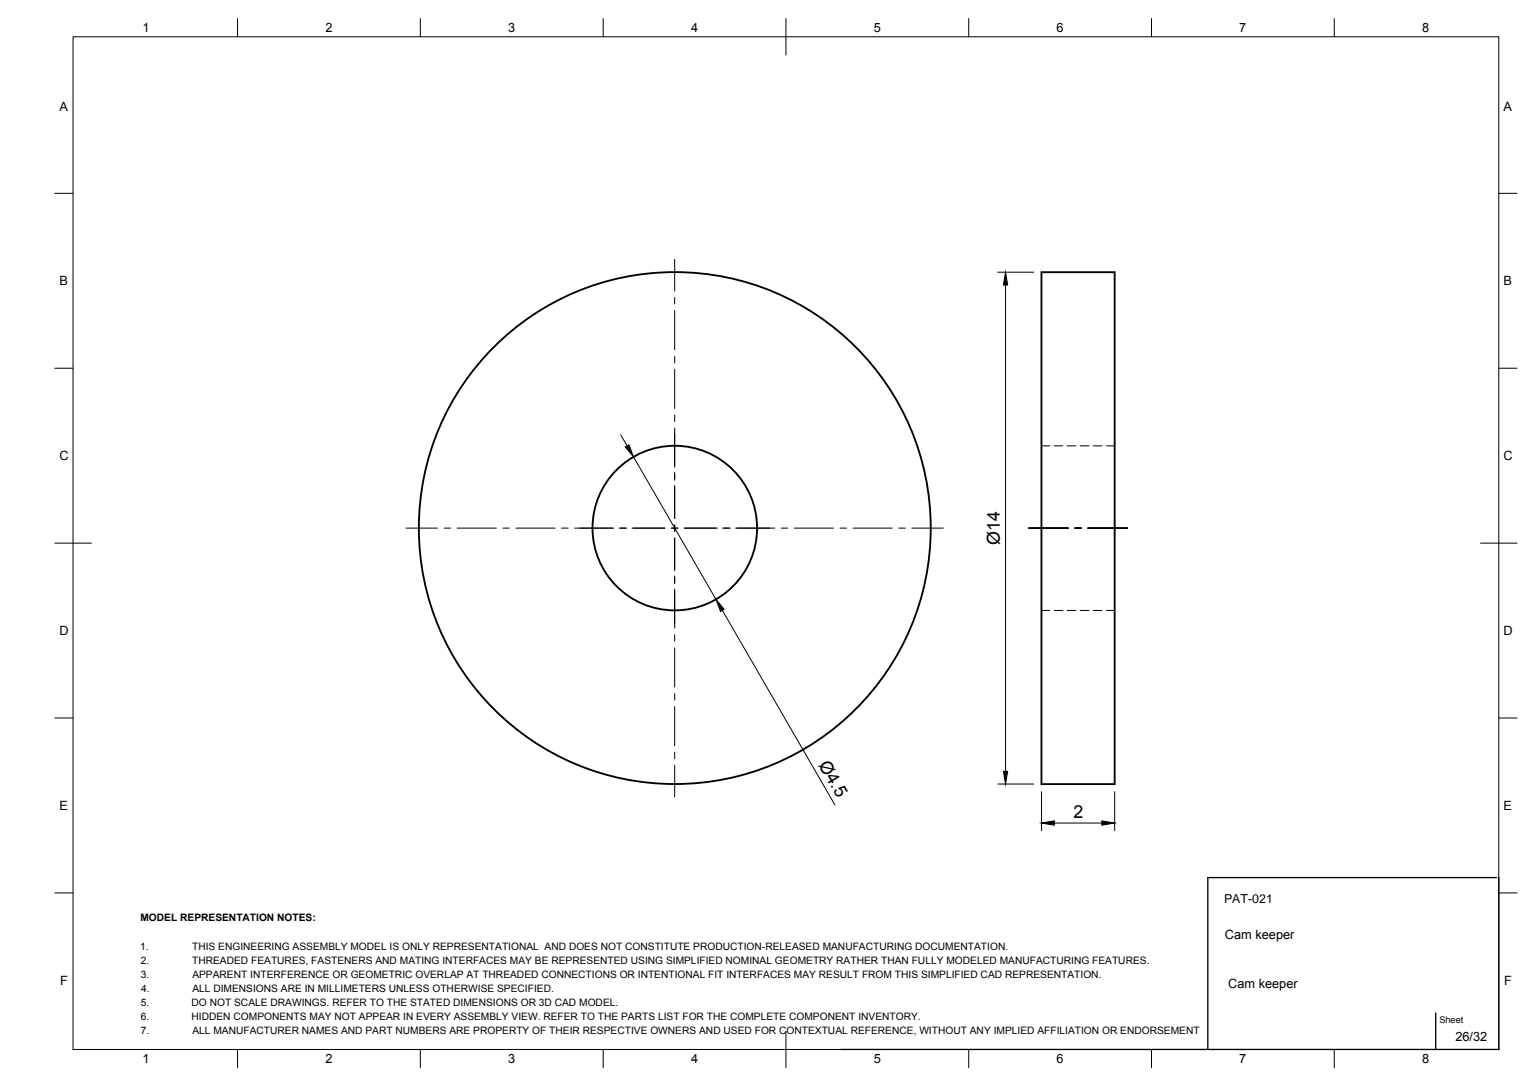
ISO-10303-21;
HEADER;
/* Generated by software containing ST-Developer
 * from STEP Tools, Inc. (www.steptools.com) 
 */

FILE_DESCRIPTION(
/* description */ ('Chain-less indexing wheel (Geneva) drive'),
/* implementation_level */ '2;1');

FILE_NAME(
/* name */ 'Cam keeper.step',
/* time_stamp */ '2026-10-28T03:25:22-07:00',
/* author */ (''),
/* organization */ (''),
/* preprocessor_version */ 'ST-DEVELOPER v20.2',
/* originating_system */ 'Autodesk Translation Framework v15.17.0.0',
/* authorisation */ '');

FILE_SCHEMA (('AUTOMOTIVE_DESIGN { 1 0 10303 214 3 1 1 }'));
ENDSEC;

DATA;
#10=MECHANICAL_DESIGN_GEOMETRIC_PRESENTATION_REPRESENTATION('',(#329),#10957);
#271=SHAPE_REPRESENTATION_RELATIONSHIP('SRR','None',#11086,#296);
#296=ADVANCED_BREP_SHAPE_REPRESENTATION('',(#361),#10949);
#329=STYLED_ITEM('',(#11273),#361);
#361=MANIFOLD_SOLID_BREP('Body1',#5726);
#451=FACE_BOUND('',#1299,.T.);
#452=FACE_BOUND('',#1301,.T.);
#585=PLANE('',#6514);
#586=PLANE('',#6515);
#879=FACE_OUTER_BOUND('',#1296,.T.);
#880=FACE_OUTER_BOUND('',#1297,.T.);
#881=FACE_OUTER_BOUND('',#1298,.T.);
#882=FACE_OUTER_BOUND('',#1300,.T.);
#1296=EDGE_LOOP('',(#4719,#4720,#4721,#4722));
#1297=EDGE_LOOP('',(#4723,#4724,#4725,#4726));
#1298=EDGE_LOOP('',(#4727));
#1299=EDGE_LOOP('',(#4728));
#1300=EDGE_LOOP('',(#4729));
#1301=EDGE_LOOP('',(#4730));
#1636=LINE('',#10193,#2010);
#1637=LINE('',#10199,#2011);
#2010=VECTOR('',#7962,0.225);
#2011=VECTOR('',#7969,0.7);
#2414=CIRCLE('',#6509,0.225);
#2415=CIRCLE('',#6510,0.225);
#2416=CIRCLE('',#6512,0.7);
#2417=CIRCLE('',#6513,0.7);
#2826=VERTEX_POINT('',#10190);
#2827=VERTEX_POINT('',#10192);
#2828=VERTEX_POINT('',#10196);
#2829=VERTEX_POINT('',#10198);
#3485=EDGE_CURVE('',#2826,#2826,#2414,.T.);
#3486=EDGE_CURVE('',#2826,#2827,#1636,.T.);
#3487=EDGE_CURVE('',#2827,#2827,#2415,.T.);
#3488=EDGE_CURVE('',#2828,#2828,#2416,.T.);
#3489=EDGE_CURVE('',#2828,#2829,#1637,.T.);
#3490=EDGE_CURVE('',#2829,#2829,#2417,.T.);
#4719=ORIENTED_EDGE('',*,*,#3485,.F.);
#4720=ORIENTED_EDGE('',*,*,#3486,.T.);
#4721=ORIENTED_EDGE('',*,*,#3487,.T.);
#4722=ORIENTED_EDGE('',*,*,#3486,.F.);
#4723=ORIENTED_EDGE('',*,*,#3488,.F.);
#4724=ORIENTED_EDGE('',*,*,#3489,.T.);
#4725=ORIENTED_EDGE('',*,*,#3490,.T.);
#4726=ORIENTED_EDGE('',*,*,#3489,.F.);
#4727=ORIENTED_EDGE('',*,*,#3488,.T.);
#4728=ORIENTED_EDGE('',*,*,#3485,.T.);
#4729=ORIENTED_EDGE('',*,*,#3490,.F.);
#4730=ORIENTED_EDGE('',*,*,#3487,.F.);
#5331=CYLINDRICAL_SURFACE('',#6508,0.225);
#5332=CYLINDRICAL_SURFACE('',#6511,0.7);
#5593=ADVANCED_FACE('',(#879),#5331,.F.);
#5594=ADVANCED_FACE('',(#880),#5332,.T.);
#5595=ADVANCED_FACE('',(#881,#451),#585,.T.);
#5596=ADVANCED_FACE('',(#882,#452),#586,.F.);
#5726=CLOSED_SHELL('',(#5593,#5594,#5595,#5596));
#6507=AXIS2_PLACEMENT_3D('',#10188,#7956,#7957);
#6508=AXIS2_PLACEMENT_3D('',#10189,#7958,#7959);
#6509=AXIS2_PLACEMENT_3D('',#10191,#7960,#7961);
#6510=AXIS2_PLACEMENT_3D('',#10194,#7963,#7964);
#6511=AXIS2_PLACEMENT_3D('',#10195,#7965,#7966);
#6512=AXIS2_PLACEMENT_3D('',#10197,#7967,#7968);
#6513=AXIS2_PLACEMENT_3D('',#10200,#7970,#7971);
#6514=AXIS2_PLACEMENT_3D('',#10201,#7972,#7973);
#6515=AXIS2_PLACEMENT_3D('',#10202,#7974,#7975);
#7956=DIRECTION('axis',(0.,0.,1.));
#7957=DIRECTION('refdir',(1.,0.,0.));
#7958=DIRECTION('center_axis',(0.,0.,1.));
#7959=DIRECTION('ref_axis',(1.,0.,0.));
#7960=DIRECTION('center_axis',(0.,0.,-1.));
#7961=DIRECTION('ref_axis',(1.,0.,0.));
#7962=DIRECTION('',(0.,0.,-1.));
#7963=DIRECTION('center_axis',(0.,0.,-1.));
#7964=DIRECTION('ref_axis',(1.,0.,0.));
#7965=DIRECTION('center_axis',(0.,0.,1.));
#7966=DIRECTION('ref_axis',(1.,0.,0.));
#7967=DIRECTION('center_axis',(0.,0.,1.));
#7968=DIRECTION('ref_axis',(1.,0.,0.));
#7969=DIRECTION('',(0.,0.,-1.));
#7970=DIRECTION('center_axis',(0.,0.,1.));
#7971=DIRECTION('ref_axis',(1.,0.,0.));
#7972=DIRECTION('center_axis',(0.,0.,1.));
#7973=DIRECTION('ref_axis',(1.,0.,0.));
#7974=DIRECTION('center_axis',(0.,0.,1.));
#7975=DIRECTION('ref_axis',(1.,0.,0.));
#10188=CARTESIAN_POINT('',(0.,0.,0.));
#10189=CARTESIAN_POINT('Origin',(0.,0.,6.8));
#10190=CARTESIAN_POINT('',(-0.225,-2.75545529808154E-17,7.));
#10191=CARTESIAN_POINT('Origin',(0.,0.,7.));
#10192=CARTESIAN_POINT('',(-0.225,-2.75545529808154E-17,6.8));
#10193=CARTESIAN_POINT('',(-0.225,-2.75545529808154E-17,6.8));
#10194=CARTESIAN_POINT('Origin',(0.,0.,6.8));
#10195=CARTESIAN_POINT('Origin',(0.,0.,6.8));
#10196=CARTESIAN_POINT('',(-0.7,-8.57252759403147E-17,7.));
#10197=CARTESIAN_POINT('Origin',(0.,0.,7.));
#10198=CARTESIAN_POINT('',(-0.7,-8.57252759403147E-17,6.8));
#10199=CARTESIAN_POINT('',(-0.7,-8.57252759403147E-17,6.8));
#10200=CARTESIAN_POINT('Origin',(0.,0.,6.8));
#10201=CARTESIAN_POINT('Origin',(0.,0.,7.));
#10202=CARTESIAN_POINT('Origin',(0.,0.,6.8));
#10918=UNCERTAINTY_MEASURE_WITH_UNIT(LENGTH_MEASURE(0.001),#10958,
'DISTANCE_ACCURACY_VALUE',
'Maximum model space distance between geometric entities at asserted c
onnectivities');
#10926=UNCERTAINTY_MEASURE_WITH_UNIT(LENGTH_MEASURE(0.001),#10958,
'DISTANCE_ACCURACY_VALUE',
'Maximum model space distance between geometric entities at asserted c
onnectivities');
#10949=(
GEOMETRIC_REPRESENTATION_CONTEXT(3)
GLOBAL_UNCERTAINTY_ASSIGNED_CONTEXT((#10918))
GLOBAL_UNIT_ASSIGNED_CONTEXT((#10958,#10960,#10961))
REPRESENTATION_CONTEXT('','3D')
);
#10957=(
GEOMETRIC_REPRESENTATION_CONTEXT(3)
GLOBAL_UNCERTAINTY_ASSIGNED_CONTEXT((#10926))
GLOBAL_UNIT_ASSIGNED_CONTEXT((#10958,#10960,#10961))
REPRESENTATION_CONTEXT('','3D')
);
#10958=(
LENGTH_UNIT()
NAMED_UNIT(*)
SI_UNIT(.CENTI.,.METRE.)
);
#10960=(
NAMED_UNIT(*)
PLANE_ANGLE_UNIT()
SI_UNIT($,.RADIAN.)
);
#10961=(
NAMED_UNIT(*)
SI_UNIT($,.STERADIAN.)
SOLID_ANGLE_UNIT()
);
#10984=SHAPE_DEFINITION_REPRESENTATION(#11019,#11086);
#11019=PRODUCT_DEFINITION_SHAPE('',$,#11117);
#11086=SHAPE_REPRESENTATION('',(#6507),#10949);
#11094=PRODUCT_DEFINITION_CONTEXT('part definition',#11186,'design');
#11117=PRODUCT_DEFINITION('Cam keeper','Cam keeper',#11147,#11094);
#11147=PRODUCT_DEFINITION_FORMATION('',$,#11210);
#11186=APPLICATION_CONTEXT(
'Core Data for Automotive Mechanical Design Process');
#11187=PRODUCT_CONTEXT('part definition',#11186,'mechanical');
#11210=PRODUCT('Cam keeper','Cam keeper','Cam keeper',(#11187));
#11267=COLOUR_RGB('Light Blue',0.38,0.62,0.78);
#11268=FILL_AREA_STYLE_COLOUR('',#11267);
#11269=FILL_AREA_STYLE('',(#11268));
#11270=SURFACE_STYLE_FILL_AREA(#11269);
#11271=SURFACE_SIDE_STYLE('',(#11270));
#11272=SURFACE_STYLE_USAGE(.BOTH.,#11271);
#11273=PRESENTATION_STYLE_ASSIGNMENT((#11272));
ENDSEC;
END-ISO-10303-21;
